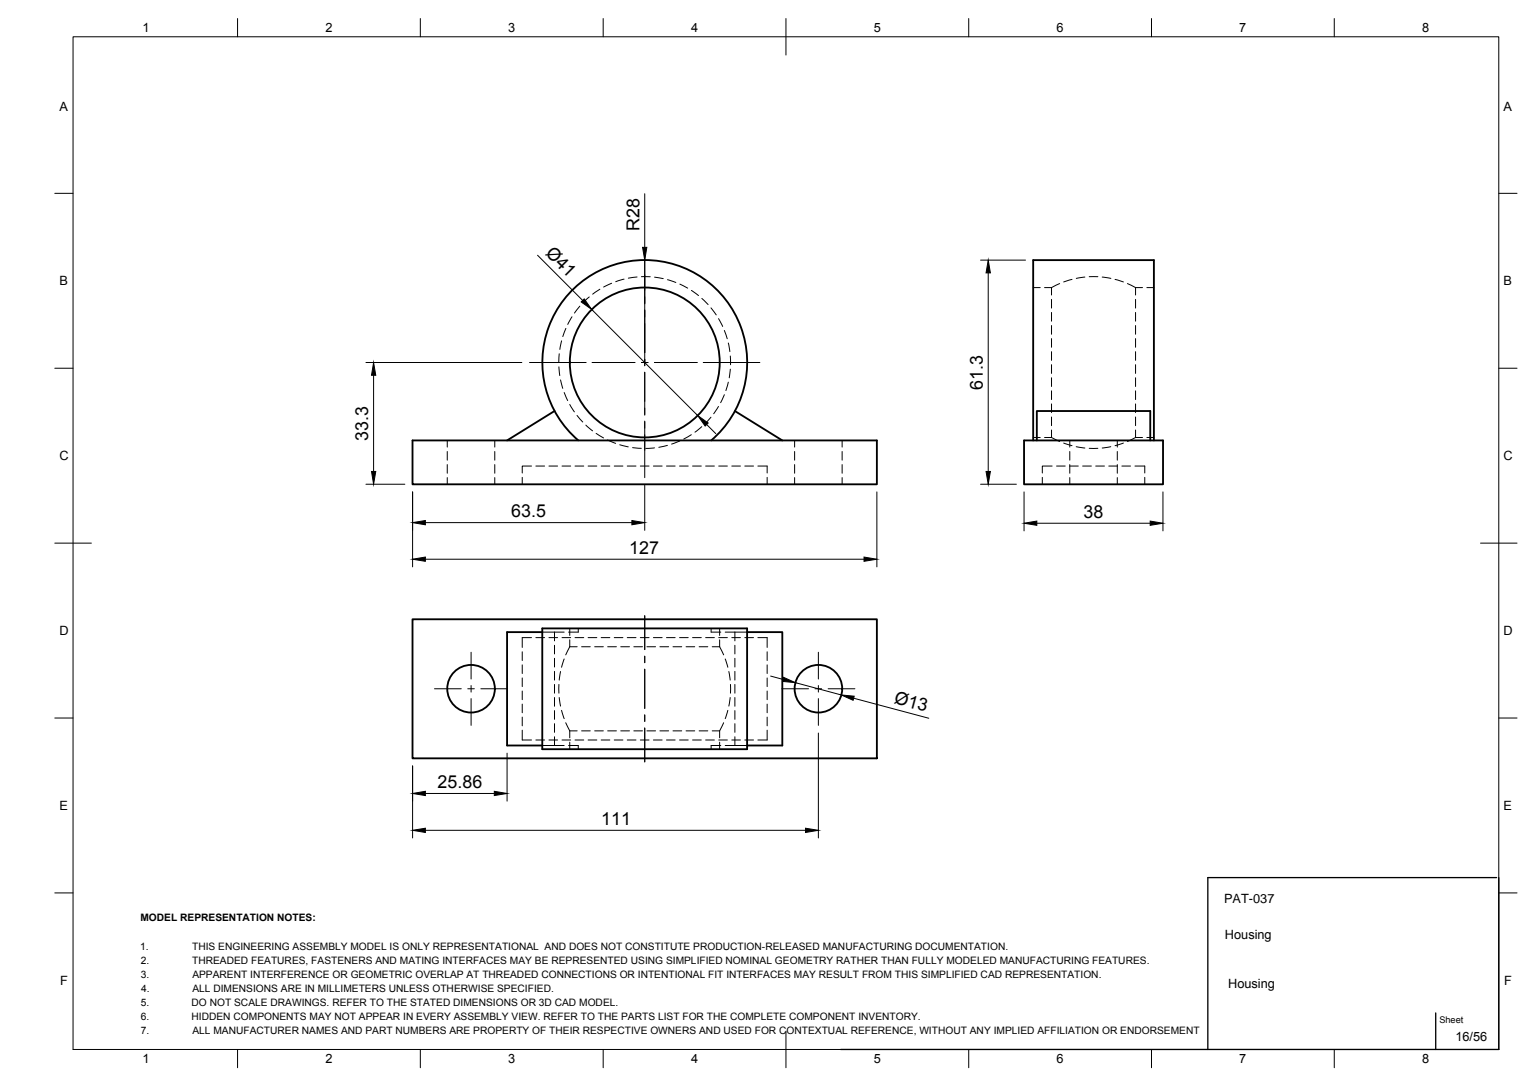
ISO-10303-21;
HEADER;
/* Generated by software containing ST-Developer
 * from STEP Tools, Inc. (www.steptools.com) 
 */

FILE_DESCRIPTION(
/* description */ ('Flywheel Crank-Slider'),
/* implementation_level */ '2;1');

FILE_NAME(
/* name */ 'Housing.step',
/* time_stamp */ '2026-10-28T03:23:13-07:00',
/* author */ (''),
/* organization */ (''),
/* preprocessor_version */ 'ST-DEVELOPER v20.2',
/* originating_system */ 'Autodesk Translation Framework v15.17.0.0',
/* authorisation */ '');

FILE_SCHEMA (('AUTOMOTIVE_DESIGN { 1 0 10303 214 3 1 1 }'));
ENDSEC;

DATA;
#10=MECHANICAL_DESIGN_GEOMETRIC_PRESENTATION_REPRESENTATION('',(#680),#17322);
#511=SPHERICAL_SURFACE('',#9980,2.35);
#576=SHAPE_REPRESENTATION_RELATIONSHIP('SRR','None',#17573,#628);
#628=ADVANCED_BREP_SHAPE_REPRESENTATION('',(#740),#17277);
#680=STYLED_ITEM('',(#17910),#740);
#740=MANIFOLD_SOLID_BREP('Body1',#9059);
#862=FACE_BOUND('',#2084,.T.);
#863=FACE_BOUND('',#2085,.T.);
#864=FACE_BOUND('',#2093,.T.);
#865=FACE_BOUND('',#2094,.T.);
#866=FACE_BOUND('',#2095,.T.);
#867=FACE_BOUND('',#2098,.T.);
#868=FACE_BOUND('',#2100,.T.);
#869=FACE_BOUND('',#2113,.T.);
#870=FACE_BOUND('',#2114,.T.);
#871=FACE_BOUND('',#2115,.T.);
#1096=PLANE('',#9982);
#1097=PLANE('',#9984);
#1098=PLANE('',#9986);
#1099=PLANE('',#9988);
#1100=PLANE('',#9989);
#1101=PLANE('',#9991);
#1102=PLANE('',#9992);
#1103=PLANE('',#9998);
#1104=PLANE('',#9999);
#1105=PLANE('',#10000);
#1106=PLANE('',#10001);
#1107=PLANE('',#10002);
#1108=PLANE('',#10003);
#1109=PLANE('',#10004);
#1110=PLANE('',#10009);
#1111=PLANE('',#10010);
#1112=PLANE('',#10011);
#1113=PLANE('',#10012);
#1114=PLANE('',#10013);
#1469=FACE_OUTER_BOUND('',#2081,.T.);
#1470=FACE_OUTER_BOUND('',#2082,.T.);
#1471=FACE_OUTER_BOUND('',#2083,.T.);
#1472=FACE_OUTER_BOUND('',#2086,.T.);
#1473=FACE_OUTER_BOUND('',#2087,.T.);
#1474=FACE_OUTER_BOUND('',#2088,.T.);
#1475=FACE_OUTER_BOUND('',#2089,.T.);
#1476=FACE_OUTER_BOUND('',#2090,.T.);
#1477=FACE_OUTER_BOUND('',#2091,.T.);
#1478=FACE_OUTER_BOUND('',#2092,.T.);
#1479=FACE_OUTER_BOUND('',#2096,.T.);
#1480=FACE_OUTER_BOUND('',#2097,.T.);
#1481=FACE_OUTER_BOUND('',#2099,.T.);
#1482=FACE_OUTER_BOUND('',#2101,.T.);
#1483=FACE_OUTER_BOUND('',#2102,.T.);
#1484=FACE_OUTER_BOUND('',#2103,.T.);
#1485=FACE_OUTER_BOUND('',#2104,.T.);
#1486=FACE_OUTER_BOUND('',#2105,.T.);
#1487=FACE_OUTER_BOUND('',#2106,.T.);
#1488=FACE_OUTER_BOUND('',#2107,.T.);
#1489=FACE_OUTER_BOUND('',#2108,.T.);
#1490=FACE_OUTER_BOUND('',#2109,.T.);
#1491=FACE_OUTER_BOUND('',#2110,.T.);
#1492=FACE_OUTER_BOUND('',#2111,.T.);
#1493=FACE_OUTER_BOUND('',#2112,.T.);
#2081=EDGE_LOOP('',(#6718,#6719,#6720,#6721));
#2082=EDGE_LOOP('',(#6722,#6723,#6724,#6725));
#2083=EDGE_LOOP('',(#6726,#6727));
#2084=EDGE_LOOP('',(#6728));
#2085=EDGE_LOOP('',(#6729));
#2086=EDGE_LOOP('',(#6730,#6731,#6732));
#2087=EDGE_LOOP('',(#6733,#6734,#6735));
#2088=EDGE_LOOP('',(#6736,#6737,#6738));
#2089=EDGE_LOOP('',(#6739,#6740,#6741,#6742));
#2090=EDGE_LOOP('',(#6743,#6744,#6745));
#2091=EDGE_LOOP('',(#6746,#6747,#6748,#6749));
#2092=EDGE_LOOP('',(#6750,#6751,#6752,#6753));
#2093=EDGE_LOOP('',(#6754));
#2094=EDGE_LOOP('',(#6755));
#2095=EDGE_LOOP('',(#6756,#6757,#6758,#6759,#6760,#6761,#6762,#6763,#6764,
#6765,#6766,#6767));
#2096=EDGE_LOOP('',(#6768,#6769,#6770,#6771,#6772,#6773,#6774,#6775,#6776,
#6777,#6778,#6779));
#2097=EDGE_LOOP('',(#6780,#6781));
#2098=EDGE_LOOP('',(#6782));
#2099=EDGE_LOOP('',(#6783,#6784));
#2100=EDGE_LOOP('',(#6785));
#2101=EDGE_LOOP('',(#6786,#6787,#6788,#6789));
#2102=EDGE_LOOP('',(#6790,#6791,#6792,#6793));
#2103=EDGE_LOOP('',(#6794,#6795,#6796,#6797));
#2104=EDGE_LOOP('',(#6798,#6799,#6800,#6801));
#2105=EDGE_LOOP('',(#6802,#6803,#6804,#6805));
#2106=EDGE_LOOP('',(#6806,#6807,#6808,#6809));
#2107=EDGE_LOOP('',(#6810,#6811,#6812,#6813));
#2108=EDGE_LOOP('',(#6814,#6815,#6816,#6817));
#2109=EDGE_LOOP('',(#6818,#6819,#6820,#6821));
#2110=EDGE_LOOP('',(#6822,#6823,#6824,#6825));
#2111=EDGE_LOOP('',(#6826,#6827,#6828,#6829));
#2112=EDGE_LOOP('',(#6830,#6831,#6832,#6833));
#2113=EDGE_LOOP('',(#6834,#6835,#6836,#6837));
#2114=EDGE_LOOP('',(#6838));
#2115=EDGE_LOOP('',(#6839));
#2790=LINE('',#14390,#3401);
#2791=LINE('',#14396,#3402);
#2792=LINE('',#14405,#3403);
#2793=LINE('',#14407,#3404);
#2794=LINE('',#14412,#3405);
#2795=LINE('',#14415,#3406);
#2796=LINE('',#14419,#3407);
#2797=LINE('',#14422,#3408);
#2798=LINE('',#14424,#3409);
#2799=LINE('',#14425,#3410);
#2800=LINE('',#14429,#3411);
#2801=LINE('',#14431,#3412);
#2802=LINE('',#14434,#3413);
#2803=LINE('',#14435,#3414);
#2804=LINE('',#14439,#3415);
#2805=LINE('',#14441,#3416);
#2806=LINE('',#14443,#3417);
#2807=LINE('',#14444,#3418);
#2808=LINE('',#14450,#3419);
#2809=LINE('',#14452,#3420);
#2810=LINE('',#14453,#3421);
#2811=LINE('',#14455,#3422);
#2812=LINE('',#14457,#3423);
#2813=LINE('',#14458,#3424);
#2814=LINE('',#14467,#3425);
#2815=LINE('',#14469,#3426);
#2816=LINE('',#14471,#3427);
#2817=LINE('',#14472,#3428);
#2818=LINE('',#14475,#3429);
#2819=LINE('',#14477,#3430);
#2820=LINE('',#14478,#3431);
#2821=LINE('',#14481,#3432);
#2822=LINE('',#14483,#3433);
#2823=LINE('',#14484,#3434);
#2824=LINE('',#14486,#3435);
#2825=LINE('',#14487,#3436);
#2826=LINE('',#14492,#3437);
#2827=LINE('',#14496,#3438);
#2828=LINE('',#14500,#3439);
#2829=LINE('',#14501,#3440);
#2830=LINE('',#14502,#3441);
#2831=LINE('',#14505,#3442);
#2832=LINE('',#14506,#3443);
#2833=LINE('',#14509,#3444);
#2834=LINE('',#14510,#3445);
#2835=LINE('',#14512,#3446);
#3401=VECTOR('',#11586,2.05);
#3402=VECTOR('',#11593,2.05);
#3403=VECTOR('',#11602,1.);
#3404=VECTOR('',#11603,1.);
#3405=VECTOR('',#11608,1.);
#3406=VECTOR('',#11611,1.);
#3407=VECTOR('',#11614,1.);
#3408=VECTOR('',#11617,1.);
#3409=VECTOR('',#11620,1.);
#3410=VECTOR('',#11621,1.);
#3411=VECTOR('',#11624,1.);
#3412=VECTOR('',#11625,1.);
#3413=VECTOR('',#11630,1.);
#3414=VECTOR('',#11631,1.);
#3415=VECTOR('',#11634,1.);
#3416=VECTOR('',#11635,1.);
#3417=VECTOR('',#11636,1.);
#3418=VECTOR('',#11637,1.);
#3419=VECTOR('',#11642,1.);
#3420=VECTOR('',#11643,1.);
#3421=VECTOR('',#11644,1.);
#3422=VECTOR('',#11645,1.);
#3423=VECTOR('',#11646,1.);
#3424=VECTOR('',#11647,1.);
#3425=VECTOR('',#11660,1.);
#3426=VECTOR('',#11661,1.);
#3427=VECTOR('',#11662,1.);
#3428=VECTOR('',#11663,1.);
#3429=VECTOR('',#11666,1.);
#3430=VECTOR('',#11667,1.);
#3431=VECTOR('',#11668,1.);
#3432=VECTOR('',#11671,1.);
#3433=VECTOR('',#11672,1.);
#3434=VECTOR('',#11673,1.);
#3435=VECTOR('',#11676,1.);
#3436=VECTOR('',#11677,1.);
#3437=VECTOR('',#11684,0.65);
#3438=VECTOR('',#11689,0.65);
#3439=VECTOR('',#11692,1.);
#3440=VECTOR('',#11693,1.);
#3441=VECTOR('',#11694,1.);
#3442=VECTOR('',#11697,1.);
#3443=VECTOR('',#11698,1.);
#3444=VECTOR('',#11701,1.);
#3445=VECTOR('',#11702,1.);
#3446=VECTOR('',#11705,1.);
#3962=CIRCLE('',#9975,2.05);
#3963=CIRCLE('',#9976,2.05);
#3964=CIRCLE('',#9978,2.05);
#3965=CIRCLE('',#9979,2.05);
#3966=CIRCLE('',#9981,2.35);
#3967=CIRCLE('',#9983,2.8);
#3968=CIRCLE('',#9985,2.8);
#3969=CIRCLE('',#9987,2.8);
#3970=CIRCLE('',#9990,2.8);
#3971=CIRCLE('',#9993,0.65);
#3972=CIRCLE('',#9994,0.65);
#3973=CIRCLE('',#9996,2.8);
#3974=CIRCLE('',#9997,2.8);
#3975=CIRCLE('',#10006,0.65);
#3976=CIRCLE('',#10008,0.65);
#4469=VERTEX_POINT('',#14387);
#4470=VERTEX_POINT('',#14389);
#4471=VERTEX_POINT('',#14393);
#4472=VERTEX_POINT('',#14395);
#4473=VERTEX_POINT('',#14399);
#4474=VERTEX_POINT('',#14400);
#4475=VERTEX_POINT('',#14403);
#4476=VERTEX_POINT('',#14404);
#4477=VERTEX_POINT('',#14406);
#4478=VERTEX_POINT('',#14410);
#4479=VERTEX_POINT('',#14411);
#4480=VERTEX_POINT('',#14413);
#4481=VERTEX_POINT('',#14417);
#4482=VERTEX_POINT('',#14418);
#4483=VERTEX_POINT('',#14420);
#4484=VERTEX_POINT('',#14427);
#4485=VERTEX_POINT('',#14428);
#4486=VERTEX_POINT('',#14430);
#4487=VERTEX_POINT('',#14437);
#4488=VERTEX_POINT('',#14438);
#4489=VERTEX_POINT('',#14440);
#4490=VERTEX_POINT('',#14442);
#4491=VERTEX_POINT('',#14445);
#4492=VERTEX_POINT('',#14447);
#4493=VERTEX_POINT('',#14449);
#4494=VERTEX_POINT('',#14451);
#4495=VERTEX_POINT('',#14454);
#4496=VERTEX_POINT('',#14456);
#4497=VERTEX_POINT('',#14465);
#4498=VERTEX_POINT('',#14466);
#4499=VERTEX_POINT('',#14468);
#4500=VERTEX_POINT('',#14470);
#4501=VERTEX_POINT('',#14474);
#4502=VERTEX_POINT('',#14476);
#4503=VERTEX_POINT('',#14480);
#4504=VERTEX_POINT('',#14482);
#4505=VERTEX_POINT('',#14490);
#4506=VERTEX_POINT('',#14494);
#4507=VERTEX_POINT('',#14498);
#4508=VERTEX_POINT('',#14499);
#4509=VERTEX_POINT('',#14504);
#4510=VERTEX_POINT('',#14508);
#5316=EDGE_CURVE('',#4469,#4469,#3962,.T.);
#5317=EDGE_CURVE('',#4469,#4470,#2790,.T.);
#5318=EDGE_CURVE('',#4470,#4470,#3963,.T.);
#5319=EDGE_CURVE('',#4471,#4471,#3964,.T.);
#5320=EDGE_CURVE('',#4471,#4472,#2791,.T.);
#5321=EDGE_CURVE('',#4472,#4472,#3965,.T.);
#5322=EDGE_CURVE('',#4473,#4474,#3966,.T.);
#5323=EDGE_CURVE('',#4475,#4476,#2792,.T.);
#5324=EDGE_CURVE('',#4475,#4477,#2793,.T.);
#5325=EDGE_CURVE('',#4476,#4477,#3967,.T.);
#5326=EDGE_CURVE('',#4478,#4479,#2794,.T.);
#5327=EDGE_CURVE('',#4480,#4478,#3968,.T.);
#5328=EDGE_CURVE('',#4480,#4479,#2795,.T.);
#5329=EDGE_CURVE('',#4481,#4482,#2796,.T.);
#5330=EDGE_CURVE('',#4483,#4481,#3969,.T.);
#5331=EDGE_CURVE('',#4483,#4482,#2797,.T.);
#5332=EDGE_CURVE('',#4482,#4475,#2798,.T.);
#5333=EDGE_CURVE('',#4477,#4483,#2799,.T.);
#5334=EDGE_CURVE('',#4484,#4485,#2800,.T.);
#5335=EDGE_CURVE('',#4484,#4486,#2801,.T.);
#5336=EDGE_CURVE('',#4485,#4486,#3970,.T.);
#5337=EDGE_CURVE('',#4479,#4484,#2802,.T.);
#5338=EDGE_CURVE('',#4486,#4480,#2803,.T.);
#5339=EDGE_CURVE('',#4487,#4488,#2804,.T.);
#5340=EDGE_CURVE('',#4488,#4489,#2805,.T.);
#5341=EDGE_CURVE('',#4489,#4490,#2806,.T.);
#5342=EDGE_CURVE('',#4490,#4487,#2807,.T.);
#5343=EDGE_CURVE('',#4491,#4491,#3971,.T.);
#5344=EDGE_CURVE('',#4492,#4492,#3972,.T.);
#5345=EDGE_CURVE('',#4485,#4493,#2808,.T.);
#5346=EDGE_CURVE('',#4493,#4494,#2809,.T.);
#5347=EDGE_CURVE('',#4494,#4481,#2810,.T.);
#5348=EDGE_CURVE('',#4476,#4495,#2811,.T.);
#5349=EDGE_CURVE('',#4495,#4496,#2812,.T.);
#5350=EDGE_CURVE('',#4496,#4478,#2813,.T.);
#5351=EDGE_CURVE('',#4495,#4496,#3973,.T.);
#5352=EDGE_CURVE('',#4493,#4494,#3974,.T.);
#5353=EDGE_CURVE('',#4497,#4498,#2814,.T.);
#5354=EDGE_CURVE('',#4497,#4499,#2815,.T.);
#5355=EDGE_CURVE('',#4499,#4500,#2816,.T.);
#5356=EDGE_CURVE('',#4498,#4500,#2817,.T.);
#5357=EDGE_CURVE('',#4501,#4497,#2818,.T.);
#5358=EDGE_CURVE('',#4501,#4502,#2819,.T.);
#5359=EDGE_CURVE('',#4502,#4499,#2820,.T.);
#5360=EDGE_CURVE('',#4503,#4501,#2821,.T.);
#5361=EDGE_CURVE('',#4503,#4504,#2822,.T.);
#5362=EDGE_CURVE('',#4504,#4502,#2823,.T.);
#5363=EDGE_CURVE('',#4498,#4503,#2824,.T.);
#5364=EDGE_CURVE('',#4500,#4504,#2825,.T.);
#5365=EDGE_CURVE('',#4505,#4505,#3975,.T.);
#5366=EDGE_CURVE('',#4505,#4492,#2826,.T.);
#5367=EDGE_CURVE('',#4506,#4506,#3976,.T.);
#5368=EDGE_CURVE('',#4506,#4491,#2827,.T.);
#5369=EDGE_CURVE('',#4507,#4508,#2828,.T.);
#5370=EDGE_CURVE('',#4508,#4487,#2829,.T.);
#5371=EDGE_CURVE('',#4507,#4490,#2830,.T.);
#5372=EDGE_CURVE('',#4509,#4507,#2831,.T.);
#5373=EDGE_CURVE('',#4509,#4489,#2832,.T.);
#5374=EDGE_CURVE('',#4510,#4509,#2833,.T.);
#5375=EDGE_CURVE('',#4510,#4488,#2834,.T.);
#5376=EDGE_CURVE('',#4508,#4510,#2835,.T.);
#6718=ORIENTED_EDGE('',*,*,#5316,.F.);
#6719=ORIENTED_EDGE('',*,*,#5317,.T.);
#6720=ORIENTED_EDGE('',*,*,#5318,.F.);
#6721=ORIENTED_EDGE('',*,*,#5317,.F.);
#6722=ORIENTED_EDGE('',*,*,#5319,.F.);
#6723=ORIENTED_EDGE('',*,*,#5320,.T.);
#6724=ORIENTED_EDGE('',*,*,#5321,.F.);
#6725=ORIENTED_EDGE('',*,*,#5320,.F.);
#6726=ORIENTED_EDGE('',*,*,#5322,.T.);
#6727=ORIENTED_EDGE('',*,*,#5322,.F.);
#6728=ORIENTED_EDGE('',*,*,#5319,.T.);
#6729=ORIENTED_EDGE('',*,*,#5318,.T.);
#6730=ORIENTED_EDGE('',*,*,#5323,.F.);
#6731=ORIENTED_EDGE('',*,*,#5324,.T.);
#6732=ORIENTED_EDGE('',*,*,#5325,.F.);
#6733=ORIENTED_EDGE('',*,*,#5326,.F.);
#6734=ORIENTED_EDGE('',*,*,#5327,.F.);
#6735=ORIENTED_EDGE('',*,*,#5328,.T.);
#6736=ORIENTED_EDGE('',*,*,#5329,.F.);
#6737=ORIENTED_EDGE('',*,*,#5330,.F.);
#6738=ORIENTED_EDGE('',*,*,#5331,.T.);
#6739=ORIENTED_EDGE('',*,*,#5332,.F.);
#6740=ORIENTED_EDGE('',*,*,#5331,.F.);
#6741=ORIENTED_EDGE('',*,*,#5333,.F.);
#6742=ORIENTED_EDGE('',*,*,#5324,.F.);
#6743=ORIENTED_EDGE('',*,*,#5334,.F.);
#6744=ORIENTED_EDGE('',*,*,#5335,.T.);
#6745=ORIENTED_EDGE('',*,*,#5336,.F.);
#6746=ORIENTED_EDGE('',*,*,#5337,.F.);
#6747=ORIENTED_EDGE('',*,*,#5328,.F.);
#6748=ORIENTED_EDGE('',*,*,#5338,.F.);
#6749=ORIENTED_EDGE('',*,*,#5335,.F.);
#6750=ORIENTED_EDGE('',*,*,#5339,.T.);
#6751=ORIENTED_EDGE('',*,*,#5340,.T.);
#6752=ORIENTED_EDGE('',*,*,#5341,.T.);
#6753=ORIENTED_EDGE('',*,*,#5342,.T.);
#6754=ORIENTED_EDGE('',*,*,#5343,.T.);
#6755=ORIENTED_EDGE('',*,*,#5344,.T.);
#6756=ORIENTED_EDGE('',*,*,#5326,.T.);
#6757=ORIENTED_EDGE('',*,*,#5337,.T.);
#6758=ORIENTED_EDGE('',*,*,#5334,.T.);
#6759=ORIENTED_EDGE('',*,*,#5345,.T.);
#6760=ORIENTED_EDGE('',*,*,#5346,.T.);
#6761=ORIENTED_EDGE('',*,*,#5347,.T.);
#6762=ORIENTED_EDGE('',*,*,#5329,.T.);
#6763=ORIENTED_EDGE('',*,*,#5332,.T.);
#6764=ORIENTED_EDGE('',*,*,#5323,.T.);
#6765=ORIENTED_EDGE('',*,*,#5348,.T.);
#6766=ORIENTED_EDGE('',*,*,#5349,.T.);
#6767=ORIENTED_EDGE('',*,*,#5350,.T.);
#6768=ORIENTED_EDGE('',*,*,#5327,.T.);
#6769=ORIENTED_EDGE('',*,*,#5350,.F.);
#6770=ORIENTED_EDGE('',*,*,#5351,.F.);
#6771=ORIENTED_EDGE('',*,*,#5348,.F.);
#6772=ORIENTED_EDGE('',*,*,#5325,.T.);
#6773=ORIENTED_EDGE('',*,*,#5333,.T.);
#6774=ORIENTED_EDGE('',*,*,#5330,.T.);
#6775=ORIENTED_EDGE('',*,*,#5347,.F.);
#6776=ORIENTED_EDGE('',*,*,#5352,.F.);
#6777=ORIENTED_EDGE('',*,*,#5345,.F.);
#6778=ORIENTED_EDGE('',*,*,#5336,.T.);
#6779=ORIENTED_EDGE('',*,*,#5338,.T.);
#6780=ORIENTED_EDGE('',*,*,#5346,.F.);
#6781=ORIENTED_EDGE('',*,*,#5352,.T.);
#6782=ORIENTED_EDGE('',*,*,#5316,.T.);
#6783=ORIENTED_EDGE('',*,*,#5349,.F.);
#6784=ORIENTED_EDGE('',*,*,#5351,.T.);
#6785=ORIENTED_EDGE('',*,*,#5321,.T.);
#6786=ORIENTED_EDGE('',*,*,#5353,.F.);
#6787=ORIENTED_EDGE('',*,*,#5354,.T.);
#6788=ORIENTED_EDGE('',*,*,#5355,.T.);
#6789=ORIENTED_EDGE('',*,*,#5356,.F.);
#6790=ORIENTED_EDGE('',*,*,#5357,.F.);
#6791=ORIENTED_EDGE('',*,*,#5358,.T.);
#6792=ORIENTED_EDGE('',*,*,#5359,.T.);
#6793=ORIENTED_EDGE('',*,*,#5354,.F.);
#6794=ORIENTED_EDGE('',*,*,#5360,.F.);
#6795=ORIENTED_EDGE('',*,*,#5361,.T.);
#6796=ORIENTED_EDGE('',*,*,#5362,.T.);
#6797=ORIENTED_EDGE('',*,*,#5358,.F.);
#6798=ORIENTED_EDGE('',*,*,#5363,.F.);
#6799=ORIENTED_EDGE('',*,*,#5356,.T.);
#6800=ORIENTED_EDGE('',*,*,#5364,.T.);
#6801=ORIENTED_EDGE('',*,*,#5361,.F.);
#6802=ORIENTED_EDGE('',*,*,#5364,.F.);
#6803=ORIENTED_EDGE('',*,*,#5355,.F.);
#6804=ORIENTED_EDGE('',*,*,#5359,.F.);
#6805=ORIENTED_EDGE('',*,*,#5362,.F.);
#6806=ORIENTED_EDGE('',*,*,#5365,.F.);
#6807=ORIENTED_EDGE('',*,*,#5366,.T.);
#6808=ORIENTED_EDGE('',*,*,#5344,.F.);
#6809=ORIENTED_EDGE('',*,*,#5366,.F.);
#6810=ORIENTED_EDGE('',*,*,#5367,.F.);
#6811=ORIENTED_EDGE('',*,*,#5368,.T.);
#6812=ORIENTED_EDGE('',*,*,#5343,.F.);
#6813=ORIENTED_EDGE('',*,*,#5368,.F.);
#6814=ORIENTED_EDGE('',*,*,#5369,.T.);
#6815=ORIENTED_EDGE('',*,*,#5370,.T.);
#6816=ORIENTED_EDGE('',*,*,#5342,.F.);
#6817=ORIENTED_EDGE('',*,*,#5371,.F.);
#6818=ORIENTED_EDGE('',*,*,#5372,.T.);
#6819=ORIENTED_EDGE('',*,*,#5371,.T.);
#6820=ORIENTED_EDGE('',*,*,#5341,.F.);
#6821=ORIENTED_EDGE('',*,*,#5373,.F.);
#6822=ORIENTED_EDGE('',*,*,#5374,.T.);
#6823=ORIENTED_EDGE('',*,*,#5373,.T.);
#6824=ORIENTED_EDGE('',*,*,#5340,.F.);
#6825=ORIENTED_EDGE('',*,*,#5375,.F.);
#6826=ORIENTED_EDGE('',*,*,#5376,.T.);
#6827=ORIENTED_EDGE('',*,*,#5375,.T.);
#6828=ORIENTED_EDGE('',*,*,#5339,.F.);
#6829=ORIENTED_EDGE('',*,*,#5370,.F.);
#6830=ORIENTED_EDGE('',*,*,#5376,.F.);
#6831=ORIENTED_EDGE('',*,*,#5369,.F.);
#6832=ORIENTED_EDGE('',*,*,#5372,.F.);
#6833=ORIENTED_EDGE('',*,*,#5374,.F.);
#6834=ORIENTED_EDGE('',*,*,#5353,.T.);
#6835=ORIENTED_EDGE('',*,*,#5363,.T.);
#6836=ORIENTED_EDGE('',*,*,#5360,.T.);
#6837=ORIENTED_EDGE('',*,*,#5357,.T.);
#6838=ORIENTED_EDGE('',*,*,#5365,.T.);
#6839=ORIENTED_EDGE('',*,*,#5367,.T.);
#8390=CYLINDRICAL_SURFACE('',#9974,2.05);
#8391=CYLINDRICAL_SURFACE('',#9977,2.05);
#8392=CYLINDRICAL_SURFACE('',#9995,2.8);
#8393=CYLINDRICAL_SURFACE('',#10005,0.65);
#8394=CYLINDRICAL_SURFACE('',#10007,0.65);
#8660=ADVANCED_FACE('',(#1469),#8390,.F.);
#8661=ADVANCED_FACE('',(#1470),#8391,.F.);
#8662=ADVANCED_FACE('',(#1471,#862,#863),#511,.F.);
#8663=ADVANCED_FACE('',(#1472),#1096,.T.);
#8664=ADVANCED_FACE('',(#1473),#1097,.T.);
#8665=ADVANCED_FACE('',(#1474),#1098,.T.);
#8666=ADVANCED_FACE('',(#1475),#1099,.T.);
#8667=ADVANCED_FACE('',(#1476),#1100,.T.);
#8668=ADVANCED_FACE('',(#1477),#1101,.T.);
#8669=ADVANCED_FACE('',(#1478,#864,#865,#866),#1102,.T.);
#8670=ADVANCED_FACE('',(#1479),#8392,.T.);
#8671=ADVANCED_FACE('',(#1480,#867),#1103,.F.);
#8672=ADVANCED_FACE('',(#1481,#868),#1104,.T.);
#8673=ADVANCED_FACE('',(#1482),#1105,.F.);
#8674=ADVANCED_FACE('',(#1483),#1106,.F.);
#8675=ADVANCED_FACE('',(#1484),#1107,.F.);
#8676=ADVANCED_FACE('',(#1485),#1108,.F.);
#8677=ADVANCED_FACE('',(#1486),#1109,.F.);
#8678=ADVANCED_FACE('',(#1487),#8393,.F.);
#8679=ADVANCED_FACE('',(#1488),#8394,.F.);
#8680=ADVANCED_FACE('',(#1489),#1110,.T.);
#8681=ADVANCED_FACE('',(#1490),#1111,.T.);
#8682=ADVANCED_FACE('',(#1491),#1112,.T.);
#8683=ADVANCED_FACE('',(#1492),#1113,.T.);
#8684=ADVANCED_FACE('',(#1493,#869,#870,#871),#1114,.F.);
#9059=CLOSED_SHELL('',(#8660,#8661,#8662,#8663,#8664,#8665,#8666,#8667,
#8668,#8669,#8670,#8671,#8672,#8673,#8674,#8675,#8676,#8677,#8678,#8679,
#8680,#8681,#8682,#8683,#8684));
#9973=AXIS2_PLACEMENT_3D('',#14385,#11580,#11581);
#9974=AXIS2_PLACEMENT_3D('',#14386,#11582,#11583);
#9975=AXIS2_PLACEMENT_3D('',#14388,#11584,#11585);
#9976=AXIS2_PLACEMENT_3D('',#14391,#11587,#11588);
#9977=AXIS2_PLACEMENT_3D('',#14392,#11589,#11590);
#9978=AXIS2_PLACEMENT_3D('',#14394,#11591,#11592);
#9979=AXIS2_PLACEMENT_3D('',#14397,#11594,#11595);
#9980=AXIS2_PLACEMENT_3D('',#14398,#11596,#11597);
#9981=AXIS2_PLACEMENT_3D('',#14401,#11598,#11599);
#9982=AXIS2_PLACEMENT_3D('',#14402,#11600,#11601);
#9983=AXIS2_PLACEMENT_3D('',#14408,#11604,#11605);
#9984=AXIS2_PLACEMENT_3D('',#14409,#11606,#11607);
#9985=AXIS2_PLACEMENT_3D('',#14414,#11609,#11610);
#9986=AXIS2_PLACEMENT_3D('',#14416,#11612,#11613);
#9987=AXIS2_PLACEMENT_3D('',#14421,#11615,#11616);
#9988=AXIS2_PLACEMENT_3D('',#14423,#11618,#11619);
#9989=AXIS2_PLACEMENT_3D('',#14426,#11622,#11623);
#9990=AXIS2_PLACEMENT_3D('',#14432,#11626,#11627);
#9991=AXIS2_PLACEMENT_3D('',#14433,#11628,#11629);
#9992=AXIS2_PLACEMENT_3D('',#14436,#11632,#11633);
#9993=AXIS2_PLACEMENT_3D('',#14446,#11638,#11639);
#9994=AXIS2_PLACEMENT_3D('',#14448,#11640,#11641);
#9995=AXIS2_PLACEMENT_3D('',#14459,#11648,#11649);
#9996=AXIS2_PLACEMENT_3D('',#14460,#11650,#11651);
#9997=AXIS2_PLACEMENT_3D('',#14461,#11652,#11653);
#9998=AXIS2_PLACEMENT_3D('',#14462,#11654,#11655);
#9999=AXIS2_PLACEMENT_3D('',#14463,#11656,#11657);
#10000=AXIS2_PLACEMENT_3D('',#14464,#11658,#11659);
#10001=AXIS2_PLACEMENT_3D('',#14473,#11664,#11665);
#10002=AXIS2_PLACEMENT_3D('',#14479,#11669,#11670);
#10003=AXIS2_PLACEMENT_3D('',#14485,#11674,#11675);
#10004=AXIS2_PLACEMENT_3D('',#14488,#11678,#11679);
#10005=AXIS2_PLACEMENT_3D('',#14489,#11680,#11681);
#10006=AXIS2_PLACEMENT_3D('',#14491,#11682,#11683);
#10007=AXIS2_PLACEMENT_3D('',#14493,#11685,#11686);
#10008=AXIS2_PLACEMENT_3D('',#14495,#11687,#11688);
#10009=AXIS2_PLACEMENT_3D('',#14497,#11690,#11691);
#10010=AXIS2_PLACEMENT_3D('',#14503,#11695,#11696);
#10011=AXIS2_PLACEMENT_3D('',#14507,#11699,#11700);
#10012=AXIS2_PLACEMENT_3D('',#14511,#11703,#11704);
#10013=AXIS2_PLACEMENT_3D('',#14513,#11706,#11707);
#11580=DIRECTION('axis',(0.,0.,1.));
#11581=DIRECTION('refdir',(1.,0.,0.));
#11582=DIRECTION('center_axis',(0.,1.,0.));
#11583=DIRECTION('ref_axis',(1.,0.,0.));
#11584=DIRECTION('center_axis',(0.,1.,0.));
#11585=DIRECTION('ref_axis',(1.,0.,0.));
#11586=DIRECTION('',(0.,1.,0.));
#11587=DIRECTION('center_axis',(0.,-1.,0.));
#11588=DIRECTION('ref_axis',(1.,0.,0.));
#11589=DIRECTION('center_axis',(0.,1.,0.));
#11590=DIRECTION('ref_axis',(1.,0.,0.));
#11591=DIRECTION('center_axis',(0.,1.,0.));
#11592=DIRECTION('ref_axis',(1.,0.,0.));
#11593=DIRECTION('',(0.,1.,0.));
#11594=DIRECTION('center_axis',(0.,-1.,0.));
#11595=DIRECTION('ref_axis',(1.,0.,0.));
#11596=DIRECTION('center_axis',(6.12323399573677E-17,0.,1.));
#11597=DIRECTION('ref_axis',(1.,0.,0.));
#11598=DIRECTION('center_axis',(-1.22464679914735E-16,1.,0.));
#11599=DIRECTION('ref_axis',(-1.,-1.22464679914735E-16,0.));
#11600=DIRECTION('center_axis',(0.,1.,0.));
#11601=DIRECTION('ref_axis',(0.,0.,1.));
#11602=DIRECTION('',(1.,0.,0.));
#11603=DIRECTION('',(0.850265146687862,0.,0.526354614616295));
#11604=DIRECTION('center_axis',(0.,1.,0.));
#11605=DIRECTION('ref_axis',(1.,0.,0.));
#11606=DIRECTION('center_axis',(0.,1.,0.));
#11607=DIRECTION('ref_axis',(0.,0.,1.));
#11608=DIRECTION('',(1.,0.,0.));
#11609=DIRECTION('center_axis',(0.,1.,0.));
#11610=DIRECTION('ref_axis',(1.,0.,0.));
#11611=DIRECTION('',(0.850265146687862,0.,-0.526354614616295));
#11612=DIRECTION('center_axis',(0.,-1.,0.));
#11613=DIRECTION('ref_axis',(0.,0.,-1.));
#11614=DIRECTION('',(-1.,0.,0.));
#11615=DIRECTION('center_axis',(0.,-1.,0.));
#11616=DIRECTION('ref_axis',(1.,0.,0.));
#11617=DIRECTION('',(-0.850265146687862,0.,-0.526354614616295));
#11618=DIRECTION('center_axis',(-0.526354614616295,0.,0.850265146687862));
#11619=DIRECTION('ref_axis',(0.850265146687862,0.,0.526354614616295));
#11620=DIRECTION('',(0.,1.,0.));
#11621=DIRECTION('',(0.,-1.,0.));
#11622=DIRECTION('center_axis',(0.,-1.,0.));
#11623=DIRECTION('ref_axis',(0.,0.,-1.));
#11624=DIRECTION('',(-1.,0.,0.));
#11625=DIRECTION('',(-0.850265146687862,0.,0.526354614616295));
#11626=DIRECTION('center_axis',(0.,-1.,0.));
#11627=DIRECTION('ref_axis',(1.,0.,0.));
#11628=DIRECTION('center_axis',(0.526354614616295,0.,0.850265146687862));
#11629=DIRECTION('ref_axis',(0.850265146687862,0.,-0.526354614616295));
#11630=DIRECTION('',(0.,-1.,0.));
#11631=DIRECTION('',(0.,1.,0.));
#11632=DIRECTION('center_axis',(0.,0.,1.));
#11633=DIRECTION('ref_axis',(1.,0.,0.));
#11634=DIRECTION('',(0.,-1.,0.));
#11635=DIRECTION('',(1.,0.,0.));
#11636=DIRECTION('',(0.,1.,0.));
#11637=DIRECTION('',(-1.,0.,0.));
#11638=DIRECTION('center_axis',(0.,0.,-1.));
#11639=DIRECTION('ref_axis',(1.,0.,0.));
#11640=DIRECTION('center_axis',(0.,0.,-1.));
#11641=DIRECTION('ref_axis',(1.,0.,0.));
#11642=DIRECTION('',(0.,-1.,0.));
#11643=DIRECTION('',(-1.,0.,0.));
#11644=DIRECTION('',(0.,1.,0.));
#11645=DIRECTION('',(0.,1.,0.));
#11646=DIRECTION('',(1.,0.,0.));
#11647=DIRECTION('',(0.,-1.,0.));
#11648=DIRECTION('center_axis',(0.,1.,0.));
#11649=DIRECTION('ref_axis',(6.12323399573677E-17,0.,1.));
#11650=DIRECTION('center_axis',(0.,1.,0.));
#11651=DIRECTION('ref_axis',(1.,0.,0.));
#11652=DIRECTION('center_axis',(0.,-1.,0.));
#11653=DIRECTION('ref_axis',(1.,0.,0.));
#11654=DIRECTION('center_axis',(0.,1.,0.));
#11655=DIRECTION('ref_axis',(1.,0.,0.));
#11656=DIRECTION('center_axis',(0.,1.,0.));
#11657=DIRECTION('ref_axis',(1.,0.,0.));
#11658=DIRECTION('center_axis',(0.,1.,0.));
#11659=DIRECTION('ref_axis',(-1.,0.,0.));
#11660=DIRECTION('',(-1.,0.,0.));
#11661=DIRECTION('',(0.,0.,1.));
#11662=DIRECTION('',(-1.,0.,0.));
#11663=DIRECTION('',(0.,0.,1.));
#11664=DIRECTION('center_axis',(1.,0.,0.));
#11665=DIRECTION('ref_axis',(0.,1.,0.));
#11666=DIRECTION('',(0.,1.,0.));
#11667=DIRECTION('',(0.,0.,1.));
#11668=DIRECTION('',(0.,1.,0.));
#11669=DIRECTION('center_axis',(0.,-1.,0.));
#11670=DIRECTION('ref_axis',(1.,0.,0.));
#11671=DIRECTION('',(1.,0.,0.));
#11672=DIRECTION('',(0.,0.,1.));
#11673=DIRECTION('',(1.,0.,0.));
#11674=DIRECTION('center_axis',(-1.,0.,0.));
#11675=DIRECTION('ref_axis',(0.,-1.,0.));
#11676=DIRECTION('',(0.,-1.,0.));
#11677=DIRECTION('',(0.,-1.,0.));
#11678=DIRECTION('center_axis',(0.,0.,1.));
#11679=DIRECTION('ref_axis',(1.,0.,0.));
#11680=DIRECTION('center_axis',(0.,0.,1.));
#11681=DIRECTION('ref_axis',(1.,0.,0.));
#11682=DIRECTION('center_axis',(0.,0.,1.));
#11683=DIRECTION('ref_axis',(1.,0.,0.));
#11684=DIRECTION('',(0.,0.,1.));
#11685=DIRECTION('center_axis',(0.,0.,1.));
#11686=DIRECTION('ref_axis',(1.,0.,0.));
#11687=DIRECTION('center_axis',(0.,0.,1.));
#11688=DIRECTION('ref_axis',(1.,0.,0.));
#11689=DIRECTION('',(0.,0.,1.));
#11690=DIRECTION('center_axis',(0.,1.,0.));
#11691=DIRECTION('ref_axis',(-1.,0.,0.));
#11692=DIRECTION('',(-1.,0.,0.));
#11693=DIRECTION('',(0.,0.,1.));
#11694=DIRECTION('',(0.,0.,1.));
#11695=DIRECTION('center_axis',(1.,0.,0.));
#11696=DIRECTION('ref_axis',(0.,1.,0.));
#11697=DIRECTION('',(0.,1.,0.));
#11698=DIRECTION('',(0.,0.,1.));
#11699=DIRECTION('center_axis',(0.,-1.,0.));
#11700=DIRECTION('ref_axis',(1.,0.,0.));
#11701=DIRECTION('',(1.,0.,0.));
#11702=DIRECTION('',(0.,0.,1.));
#11703=DIRECTION('center_axis',(-1.,0.,0.));
#11704=DIRECTION('ref_axis',(0.,-1.,0.));
#11705=DIRECTION('',(0.,-1.,0.));
#11706=DIRECTION('center_axis',(0.,0.,1.));
#11707=DIRECTION('ref_axis',(1.,0.,0.));
#14385=CARTESIAN_POINT('',(0.,0.,0.));
#14386=CARTESIAN_POINT('Origin',(0.,0.,0.));
#14387=CARTESIAN_POINT('',(-2.05,-1.65,2.51052593825207E-16));
#14388=CARTESIAN_POINT('Origin',(0.,-1.65,0.));
#14389=CARTESIAN_POINT('',(-2.05,-1.14891252930761,-2.51052593825207E-16));
#14390=CARTESIAN_POINT('',(-2.05,0.,2.51052593825207E-16));
#14391=CARTESIAN_POINT('Origin',(0.,-1.14891252930761,0.));
#14392=CARTESIAN_POINT('Origin',(0.,0.,0.));
#14393=CARTESIAN_POINT('',(-2.05,1.14891252930761,2.51052593825207E-16));
#14394=CARTESIAN_POINT('Origin',(0.,1.14891252930761,0.));
#14395=CARTESIAN_POINT('',(-2.05,1.65,-2.51052593825207E-16));
#14396=CARTESIAN_POINT('',(-2.05,0.,2.51052593825207E-16));
#14397=CARTESIAN_POINT('Origin',(0.,1.65,0.));
#14398=CARTESIAN_POINT('Origin',(0.,0.,0.));
#14399=CARTESIAN_POINT('',(-1.43895998899814E-16,-1.76221774462768E-32,
-2.35));
#14400=CARTESIAN_POINT('',(-1.43895998899814E-16,-1.76221774462768E-32,
2.35));
#14401=CARTESIAN_POINT('Origin',(0.,0.,0.));
#14402=CARTESIAN_POINT('Origin',(0.,1.55,-1.49));
#14403=CARTESIAN_POINT('',(-3.76384615384615,1.55,-2.13));
#14404=CARTESIAN_POINT('',(-1.81744325908679,1.55,-2.13));
#14405=CARTESIAN_POINT('',(0.,1.55,-2.13));
#14406=CARTESIAN_POINT('',(-2.46585583768694,1.55,-1.32648218523477));
#14407=CARTESIAN_POINT('',(-1.68,1.55,-0.84));
#14408=CARTESIAN_POINT('Origin',(0.,1.55,0.));
#14409=CARTESIAN_POINT('Origin',(0.,1.55,-1.49));
#14410=CARTESIAN_POINT('',(1.81744325908679,1.55,-2.13));
#14411=CARTESIAN_POINT('',(3.76384615384615,1.55,-2.13));
#14412=CARTESIAN_POINT('',(0.,1.55,-2.13));
#14413=CARTESIAN_POINT('',(2.46585583768694,1.55,-1.32648218523477));
#14414=CARTESIAN_POINT('Origin',(0.,1.55,0.));
#14415=CARTESIAN_POINT('',(3.78,1.55,-2.14));
#14416=CARTESIAN_POINT('Origin',(0.,-1.55,-1.49));
#14417=CARTESIAN_POINT('',(-1.81744325908679,-1.55,-2.13));
#14418=CARTESIAN_POINT('',(-3.76384615384615,-1.55,-2.13));
#14419=CARTESIAN_POINT('',(0.,-1.55,-2.13));
#14420=CARTESIAN_POINT('',(-2.46585583768694,-1.55,-1.32648218523477));
#14421=CARTESIAN_POINT('Origin',(0.,-1.55,0.));
#14422=CARTESIAN_POINT('',(-1.68,-1.55,-0.84));
#14423=CARTESIAN_POINT('Origin',(-3.78,0.,-2.14));
#14424=CARTESIAN_POINT('',(-3.76384615384615,0.,-2.13));
#14425=CARTESIAN_POINT('',(-2.46585583768694,0.,-1.32648218523477));
#14426=CARTESIAN_POINT('Origin',(0.,-1.55,-1.49));
#14427=CARTESIAN_POINT('',(3.76384615384615,-1.55,-2.13));
#14428=CARTESIAN_POINT('',(1.81744325908679,-1.55,-2.13));
#14429=CARTESIAN_POINT('',(0.,-1.55,-2.13));
#14430=CARTESIAN_POINT('',(2.46585583768694,-1.55,-1.32648218523477));
#14431=CARTESIAN_POINT('',(3.78,-1.55,-2.14));
#14432=CARTESIAN_POINT('Origin',(0.,-1.55,0.));
#14433=CARTESIAN_POINT('Origin',(1.68,0.,-0.84));
#14434=CARTESIAN_POINT('',(3.76384615384615,0.,-2.13));
#14435=CARTESIAN_POINT('',(2.46585583768694,0.,-1.32648218523477));
#14436=CARTESIAN_POINT('Origin',(0.,0.,-2.13));
#14437=CARTESIAN_POINT('',(-6.35,1.9,-2.13));
#14438=CARTESIAN_POINT('',(-6.35,-1.9,-2.13));
#14439=CARTESIAN_POINT('',(-6.35,1.9,-2.13));
#14440=CARTESIAN_POINT('',(6.35,-1.9,-2.13));
#14441=CARTESIAN_POINT('',(-6.35,-1.9,-2.13));
#14442=CARTESIAN_POINT('',(6.35,1.9,-2.13));
#14443=CARTESIAN_POINT('',(6.35,-1.9,-2.13));
#14444=CARTESIAN_POINT('',(6.35,1.9,-2.13));
#14445=CARTESIAN_POINT('',(4.1,7.9602041944578E-17,-2.13));
#14446=CARTESIAN_POINT('Origin',(4.75,0.,-2.13));
#14447=CARTESIAN_POINT('',(-5.4,7.9602041944578E-17,-2.13));
#14448=CARTESIAN_POINT('Origin',(-4.75,0.,-2.13));
#14449=CARTESIAN_POINT('',(1.81744325908679,-1.65,-2.13));
#14450=CARTESIAN_POINT('',(1.81744325908679,0.,-2.13));
#14451=CARTESIAN_POINT('',(-1.81744325908679,-1.65,-2.13));
#14452=CARTESIAN_POINT('',(0.,-1.65,-2.13));
#14453=CARTESIAN_POINT('',(-1.81744325908679,0.,-2.13));
#14454=CARTESIAN_POINT('',(-1.81744325908679,1.65,-2.13));
#14455=CARTESIAN_POINT('',(-1.81744325908679,0.,-2.13));
#14456=CARTESIAN_POINT('',(1.81744325908679,1.65,-2.13));
#14457=CARTESIAN_POINT('',(0.,1.65,-2.13));
#14458=CARTESIAN_POINT('',(1.81744325908679,0.,-2.13));
#14459=CARTESIAN_POINT('Origin',(0.,0.,0.));
#14460=CARTESIAN_POINT('Origin',(0.,1.65,0.));
#14461=CARTESIAN_POINT('Origin',(0.,-1.65,0.));
#14462=CARTESIAN_POINT('Origin',(0.,-1.65,0.));
#14463=CARTESIAN_POINT('Origin',(0.,1.65,0.));
#14464=CARTESIAN_POINT('Origin',(3.35,1.4,-3.33));
#14465=CARTESIAN_POINT('',(3.35,1.4,-3.33));
#14466=CARTESIAN_POINT('',(-3.35,1.4,-3.33));
#14467=CARTESIAN_POINT('',(1.675,1.4,-3.33));
#14468=CARTESIAN_POINT('',(3.35,1.4,-2.83));
#14469=CARTESIAN_POINT('',(3.35,1.4,-3.33));
#14470=CARTESIAN_POINT('',(-3.35,1.4,-2.83));
#14471=CARTESIAN_POINT('',(3.35,1.4,-2.83));
#14472=CARTESIAN_POINT('',(-3.35,1.4,-3.33));
#14473=CARTESIAN_POINT('Origin',(3.35,-1.4,-3.33));
#14474=CARTESIAN_POINT('',(3.35,-1.4,-3.33));
#14475=CARTESIAN_POINT('',(3.35,-0.7,-3.33));
#14476=CARTESIAN_POINT('',(3.35,-1.4,-2.83));
#14477=CARTESIAN_POINT('',(3.35,-1.4,-3.33));
#14478=CARTESIAN_POINT('',(3.35,-1.4,-2.83));
#14479=CARTESIAN_POINT('Origin',(-3.35,-1.4,-3.33));
#14480=CARTESIAN_POINT('',(-3.35,-1.4,-3.33));
#14481=CARTESIAN_POINT('',(-1.675,-1.4,-3.33));
#14482=CARTESIAN_POINT('',(-3.35,-1.4,-2.83));
#14483=CARTESIAN_POINT('',(-3.35,-1.4,-3.33));
#14484=CARTESIAN_POINT('',(-3.35,-1.4,-2.83));
#14485=CARTESIAN_POINT('Origin',(-3.35,1.4,-3.33));
#14486=CARTESIAN_POINT('',(-3.35,0.7,-3.33));
#14487=CARTESIAN_POINT('',(-3.35,1.4,-2.83));
#14488=CARTESIAN_POINT('Origin',(0.,0.,-2.83));
#14489=CARTESIAN_POINT('Origin',(-4.75,0.,-3.33));
#14490=CARTESIAN_POINT('',(-5.4,-7.9602041944578E-17,-3.33));
#14491=CARTESIAN_POINT('Origin',(-4.75,0.,-3.33));
#14492=CARTESIAN_POINT('',(-5.4,-7.9602041944578E-17,-3.33));
#14493=CARTESIAN_POINT('Origin',(4.75,0.,-3.33));
#14494=CARTESIAN_POINT('',(4.1,-7.9602041944578E-17,-3.33));
#14495=CARTESIAN_POINT('Origin',(4.75,0.,-3.33));
#14496=CARTESIAN_POINT('',(4.1,-7.9602041944578E-17,-3.33));
#14497=CARTESIAN_POINT('Origin',(6.35,1.9,-3.33));
#14498=CARTESIAN_POINT('',(6.35,1.9,-3.33));
#14499=CARTESIAN_POINT('',(-6.35,1.9,-3.33));
#14500=CARTESIAN_POINT('',(6.35,1.9,-3.33));
#14501=CARTESIAN_POINT('',(-6.35,1.9,-3.33));
#14502=CARTESIAN_POINT('',(6.35,1.9,-3.33));
#14503=CARTESIAN_POINT('Origin',(6.35,-1.9,-3.33));
#14504=CARTESIAN_POINT('',(6.35,-1.9,-3.33));
#14505=CARTESIAN_POINT('',(6.35,-1.9,-3.33));
#14506=CARTESIAN_POINT('',(6.35,-1.9,-3.33));
#14507=CARTESIAN_POINT('Origin',(-6.35,-1.9,-3.33));
#14508=CARTESIAN_POINT('',(-6.35,-1.9,-3.33));
#14509=CARTESIAN_POINT('',(-6.35,-1.9,-3.33));
#14510=CARTESIAN_POINT('',(-6.35,-1.9,-3.33));
#14511=CARTESIAN_POINT('Origin',(-6.35,1.9,-3.33));
#14512=CARTESIAN_POINT('',(-6.35,1.9,-3.33));
#14513=CARTESIAN_POINT('Origin',(0.,0.,-3.33));
#17216=UNCERTAINTY_MEASURE_WITH_UNIT(LENGTH_MEASURE(0.001),#17323,
'DISTANCE_ACCURACY_VALUE',
'Maximum model space distance between geometric entities at asserted c
onnectivities');
#17261=UNCERTAINTY_MEASURE_WITH_UNIT(LENGTH_MEASURE(0.001),#17323,
'DISTANCE_ACCURACY_VALUE',
'Maximum model space distance between geometric entities at asserted c
onnectivities');
#17277=(
GEOMETRIC_REPRESENTATION_CONTEXT(3)
GLOBAL_UNCERTAINTY_ASSIGNED_CONTEXT((#17216))
GLOBAL_UNIT_ASSIGNED_CONTEXT((#17323,#17325,#17326))
REPRESENTATION_CONTEXT('','3D')
);
#17322=(
GEOMETRIC_REPRESENTATION_CONTEXT(3)
GLOBAL_UNCERTAINTY_ASSIGNED_CONTEXT((#17261))
GLOBAL_UNIT_ASSIGNED_CONTEXT((#17323,#17325,#17326))
REPRESENTATION_CONTEXT('','3D')
);
#17323=(
LENGTH_UNIT()
NAMED_UNIT(*)
SI_UNIT(.CENTI.,.METRE.)
);
#17325=(
NAMED_UNIT(*)
PLANE_ANGLE_UNIT()
SI_UNIT($,.RADIAN.)
);
#17326=(
NAMED_UNIT(*)
SI_UNIT($,.STERADIAN.)
SOLID_ANGLE_UNIT()
);
#17342=SHAPE_DEFINITION_REPRESENTATION(#17402,#17573);
#17402=PRODUCT_DEFINITION_SHAPE('',$,#17634);
#17573=SHAPE_REPRESENTATION('',(#9973),#17277);
#17618=PRODUCT_DEFINITION_CONTEXT('part definition',#17800,'design');
#17634=PRODUCT_DEFINITION('Housing','Housing',#17694,#17618);
#17694=PRODUCT_DEFINITION_FORMATION('',$,#17817);
#17800=APPLICATION_CONTEXT(
'Core Data for Automotive Mechanical Design Process');
#17801=PRODUCT_CONTEXT('part definition',#17800,'mechanical');
#17817=PRODUCT('Housing','Housing','Housing',(#17801));
#17904=COLOUR_RGB('Dark Blue',0.08,0.2,0.34);
#17905=FILL_AREA_STYLE_COLOUR('',#17904);
#17906=FILL_AREA_STYLE('',(#17905));
#17907=SURFACE_STYLE_FILL_AREA(#17906);
#17908=SURFACE_SIDE_STYLE('',(#17907));
#17909=SURFACE_STYLE_USAGE(.BOTH.,#17908);
#17910=PRESENTATION_STYLE_ASSIGNMENT((#17909));
ENDSEC;
END-ISO-10303-21;
